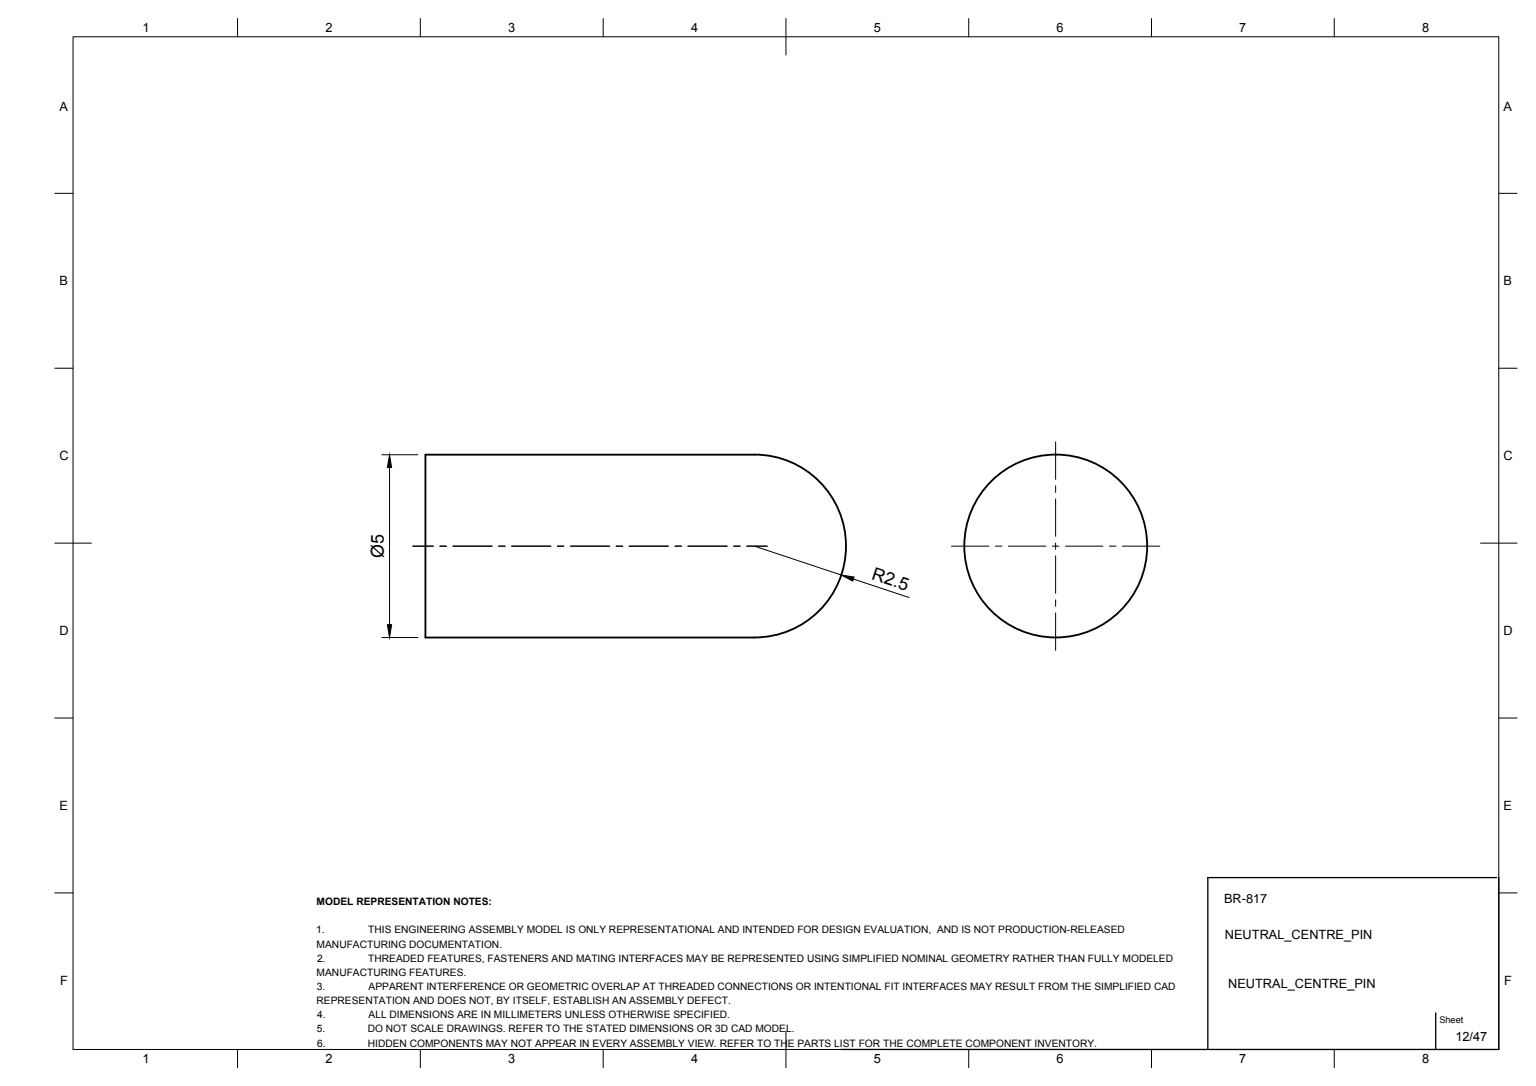
ISO-10303-21;
HEADER;
FILE_DESCRIPTION((''),'2;1');
FILE_NAME('NEUTRAL_CENTRE_PIN.step','2026-10-01T22:07:29-07:00',(''),(''),'','','');
FILE_SCHEMA (('AUTOMOTIVE_DESIGN { 1 0 10303 214 3 1 1 }'));
ENDSEC;
DATA;
#10=MECHANICAL_DESIGN_GEOMETRIC_PRESENTATION_REPRESENTATION('',(#548),#15484);
#192=SPHERICAL_SURFACE('',#8859,0.25) ;
#478=SHAPE_REPRESENTATION_RELATIONSHIP('SRR','None',#15626,#513) ;
#513=ADVANCED_BREP_SHAPE_REPRESENTATION('',(#590),#15450) ;
#548=STYLED_ITEM('',(#15834),#590) ;
#590=MANIFOLD_SOLID_BREP('NEUTRAL_CENTRE_PIN',#8257) ;
#656=CYLINDRICAL_SURFACE('',#8862,0.25) ;
#945=CIRCLE('',#8860,0.25) ;
#946=CIRCLE('',#8861,0.25) ;
#947=CIRCLE('',#8863,0.25) ;
#1471=FACE_OUTER_BOUND('',#2010,.T.) ;
#1472=FACE_OUTER_BOUND('',#2011,.T.) ;
#1473=FACE_OUTER_BOUND('',#2012,.T.) ;
#2010=EDGE_LOOP('',(#5735,#5736,#5737)) ;
#2011=EDGE_LOOP('',(#5738,#5739,#5740,#5741)) ;
#2012=EDGE_LOOP('',(#5742)) ;
#2611=LINE('',#13395,#3085) ;
#3085=VECTOR('',#10460,0.25) ;
#3542=VERTEX_POINT('',#13388) ;
#3543=VERTEX_POINT('',#13390) ;
#3544=VERTEX_POINT('',#13393) ;
#4372=EDGE_CURVE('',#3542,#3542,#945,.T.) ;
#4373=EDGE_CURVE('',#3542,#3543,#946,.T.) ;
#4374=EDGE_CURVE('',#3544,#3544,#947,.T.) ;
#4375=EDGE_CURVE('',#3544,#3542,#2611,.T.) ;
#5735=ORIENTED_EDGE('',*,*,#4372,.T.) ;
#5736=ORIENTED_EDGE('',*,*,#4373,.T.) ;
#5737=ORIENTED_EDGE('',*,*,#4373,.F.) ;
#5738=ORIENTED_EDGE('',*,*,#4374,.F.) ;
#5739=ORIENTED_EDGE('',*,*,#4375,.T.) ;
#5740=ORIENTED_EDGE('',*,*,#4372,.F.) ;
#5741=ORIENTED_EDGE('',*,*,#4375,.F.) ;
#5742=ORIENTED_EDGE('',*,*,#4374,.T.) ;
#7613=PLANE('',#8864) ;
#7858=ADVANCED_FACE('',(#1471),#192,.T.) ;
#7859=ADVANCED_FACE('',(#1472),#656,.T.) ;
#7860=ADVANCED_FACE('',(#1473),#7613,.T.) ;
#8257=CLOSED_SHELL('',(#7858,#7859,#7860)) ;
#8858=AXIS2_PLACEMENT_3D('',#13386,#10448,#10449) ;
#8859=AXIS2_PLACEMENT_3D('',#13387,#10450,#10451) ;
#8860=AXIS2_PLACEMENT_3D('',#13389,#10452,#10453) ;
#8861=AXIS2_PLACEMENT_3D('',#13391,#10454,#10455) ;
#8862=AXIS2_PLACEMENT_3D('',#13392,#10456,#10457) ;
#8863=AXIS2_PLACEMENT_3D('',#13394,#10458,#10459) ;
#8864=AXIS2_PLACEMENT_3D('',#13396,#10461,#10462) ;
#10448=DIRECTION('axis',(0.,0.,1.)) ;
#10449=DIRECTION('refdir',(1.,0.,0.)) ;
#10450=DIRECTION('center_axis',(0.,0.,1.)) ;
#10451=DIRECTION('ref_axis',(1.,0.,0.)) ;
#10452=DIRECTION('center_axis',(0.,0.,-1.)) ;
#10453=DIRECTION('ref_axis',(1.,0.,0.)) ;
#10454=DIRECTION('center_axis',(1.22464679914735E-16,-1.,0.)) ;
#10455=DIRECTION('ref_axis',(-1.,-1.22464679914735E-16,0.)) ;
#10456=DIRECTION('center_axis',(0.,0.,1.)) ;
#10457=DIRECTION('ref_axis',(1.,0.,0.)) ;
#10458=DIRECTION('center_axis',(0.,0.,1.)) ;
#10459=DIRECTION('ref_axis',(1.,0.,0.)) ;
#10460=DIRECTION('',(0.,0.,-1.)) ;
#10461=DIRECTION('center_axis',(0.,0.,1.)) ;
#10462=DIRECTION('ref_axis',(1.,0.,0.)) ;
#13386=CARTESIAN_POINT('',(0.,0.,0.)) ;
#13387=CARTESIAN_POINT('Origin',(-1.,0.,-1.1)) ;
#13388=CARTESIAN_POINT('',(-1.25,-3.06161699786838E-17,-1.1)) ;
#13389=CARTESIAN_POINT('Origin',(-1.,0.,-1.1)) ;
#13390=CARTESIAN_POINT('',(-1.,-1.87469972832732E-33,-1.35)) ;
#13391=CARTESIAN_POINT('Origin',(-1.,0.,-1.1)) ;
#13392=CARTESIAN_POINT('Origin',(-1.,0.,-0.65)) ;
#13393=CARTESIAN_POINT('',(-1.25,-3.06161699786838E-17,-0.2)) ;
#13394=CARTESIAN_POINT('Origin',(-1.,0.,-0.2)) ;
#13395=CARTESIAN_POINT('',(-1.25,-3.06161699786838E-17,-0.65)) ;
#13396=CARTESIAN_POINT('Origin',(-1.,0.,-0.2)) ;
#15407=UNCERTAINTY_MEASURE_WITH_UNIT(LENGTH_MEASURE(0.001),#15485,
'DISTANCE_ACCURACY_VALUE',
'Maximum model space distance between geometric entities at asserted c
onnectivities') ;
#15441=UNCERTAINTY_MEASURE_WITH_UNIT(LENGTH_MEASURE(0.001),#15485,
'DISTANCE_ACCURACY_VALUE',
'Maximum model space distance between geometric entities at asserted c
onnectivities') ;
#15450=(
GEOMETRIC_REPRESENTATION_CONTEXT(3)
GLOBAL_UNCERTAINTY_ASSIGNED_CONTEXT((#15407))
GLOBAL_UNIT_ASSIGNED_CONTEXT((#15485,#15487,#15488))
REPRESENTATION_CONTEXT('','3D')
) ;
#15484=(
GEOMETRIC_REPRESENTATION_CONTEXT(3)
GLOBAL_UNCERTAINTY_ASSIGNED_CONTEXT((#15441))
GLOBAL_UNIT_ASSIGNED_CONTEXT((#15485,#15487,#15488))
REPRESENTATION_CONTEXT('','3D')
) ;
#15485=(
LENGTH_UNIT()
NAMED_UNIT(*)
SI_UNIT(.CENTI.,.METRE.)
) ;
#15487=(
NAMED_UNIT(*)
PLANE_ANGLE_UNIT()
SI_UNIT($,.RADIAN.)
) ;
#15488=(
NAMED_UNIT(*)
SI_UNIT($,.STERADIAN.)
SOLID_ANGLE_UNIT()
) ;
#15497=SHAPE_DEFINITION_REPRESENTATION(#15541,#15626) ;
#15541=PRODUCT_DEFINITION_SHAPE('',$,#15669) ;
#15626=SHAPE_REPRESENTATION('',(#8858),#15450) ;
#15660=PRODUCT_DEFINITION_CONTEXT('part definition',#15788,'design') ;
#15669=PRODUCT_DEFINITION('NEUTRAL_CENTRE_PIN',
'NEUTRAL_CENTRE_PIN',#15711,#15660) ;
#15711=PRODUCT_DEFINITION_FORMATION('',$,#15798) ;
#15788=APPLICATION_CONTEXT(
'Core Data for Automotive Mechanical Design Process') ;
#15789=PRODUCT_CONTEXT('part definition',#15788,'mechanical') ;
#15798=PRODUCT('NEUTRAL_CENTRE_PIN','NEUTRAL_CENTRE_PIN',$,(#15789)) ;
#15834=PRESENTATION_STYLE_ASSIGNMENT((#15846)) ;
#15846=SURFACE_STYLE_USAGE(.BOTH.,#15858) ;
#15858=SURFACE_SIDE_STYLE('',(#15870)) ;
#15870=SURFACE_STYLE_FILL_AREA(#15882) ;
#15882=FILL_AREA_STYLE('Brass - Polished',(#15894)) ;
#15894=FILL_AREA_STYLE_COLOUR('Brass - Polished',#15906) ;
#15906=COLOUR_RGB('Brass - Polished', 0.08235294, 0.09019608, 0.10196078) ;
ENDSEC;
END-ISO-10303-21;
